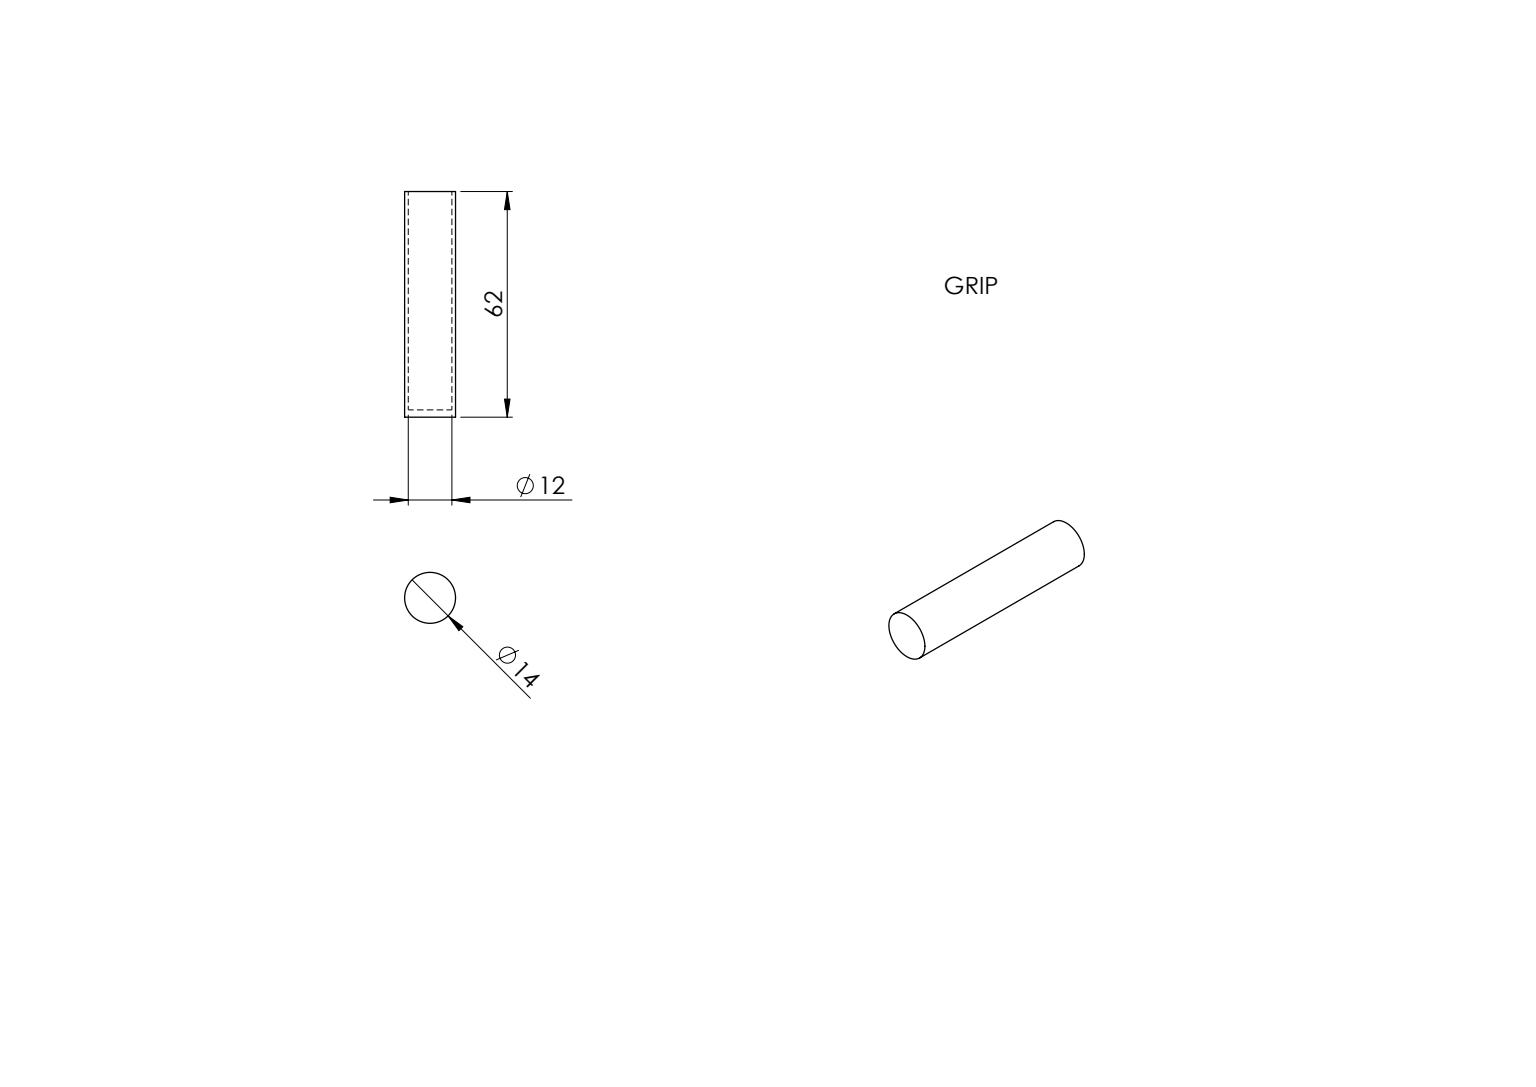
ISO-10303-21;
HEADER;
FILE_DESCRIPTION (('STEP AP214'),
    '1' );
FILE_NAME ('grip.step',
    '2026-10-25T17:17:34',
    ( '' ),
    ( '' ),
    'SwSTEP 2.0',
    'SolidWorks 2026',
    '' );
FILE_SCHEMA (( 'AUTOMOTIVE_DESIGN' ));
ENDSEC;

DATA;
#62=DIRECTION ( 'NONE',  ( -0.000000000000000000, -0.000000000000000000, -1.000000000000000000 ) ) ;
#172=ORIENTED_EDGE ( 'NONE', *, *, #15080, .F. ) ;
#270=PRODUCT_DEFINITION_CONTEXT ( 'detailed design', #8572, 'design' ) ;
#298=ORIENTED_EDGE ( 'NONE', *, *, #2474, .F. ) ;
#373=CARTESIAN_POINT ( 'NONE',  ( 118.5000000000000284, 12.69999999999998508, 50.00000000000001421 ) ) ;
#451=FACE_OUTER_BOUND ( 'NONE', #8763, .T. ) ;
#615=UNCERTAINTY_MEASURE_WITH_UNIT (LENGTH_MEASURE( 1.000000000000000082E-05 ), #15735, 'distance_accuracy_value', 'NONE');
#1092=MANIFOLD_SOLID_BREP ( 'Boss-Extrude1', #16920 ) ;
#1158=AXIS2_PLACEMENT_3D ( 'NONE', #12215, #18183, #17530 ) ;
#1175=( NAMED_UNIT ( * ) PLANE_ANGLE_UNIT ( ) SI_UNIT ( $, .RADIAN. ) );
#1608=EDGE_CURVE ( 'NONE', #14362, #14185, #5674, .T. ) ;
#1737=CIRCLE ( 'NONE', #11087, 7.000000000000006217 ) ;
#2052=SURFACE_STYLE_FILL_AREA ( #12504 ) ;
#2304=EDGE_CURVE ( 'NONE', #4985, #13752, #9705, .T. ) ;
#2362=CYLINDRICAL_SURFACE ( 'NONE', #4018, 6.000000000000005329 ) ;
#2377=AXIS2_PLACEMENT_3D ( 'NONE', #15410, #11206, #17171 ) ;
#2378=CARTESIAN_POINT ( 'NONE',  ( 111.5000000000000142, 12.69999999999998508, 50.00000000000001421 ) ) ;
#2402=VECTOR ( 'NONE', #3776, 1000.000000000000000 ) ;
#2444=FILL_AREA_STYLE_COLOUR ( '', #12359 ) ;
#2474=EDGE_CURVE ( 'NONE', #17401, #13752, #15823, .T. ) ;
#2675=ORIENTED_EDGE ( 'NONE', *, *, #1608, .F. ) ;
#2677=DIRECTION ( 'NONE',  ( 0.000000000000000000, 0.000000000000000000, 1.000000000000000000 ) ) ;
#2799=DIRECTION ( 'NONE',  ( 0.000000000000000000, 0.000000000000000000, 1.000000000000000000 ) ) ;
#2897=ORIENTED_EDGE ( 'NONE', *, *, #14345, .T. ) ;
#2959=PLANE ( 'NONE',  #16788 ) ;
#3036=CARTESIAN_POINT ( 'NONE',  ( 104.5000000000000142, 12.69999999999998508, 112.0000000000000142 ) ) ;
#3146=DIRECTION ( 'NONE',  ( 1.000000000000000000, 0.000000000000000000, -0.000000000000000000 ) ) ;
#3182=MECHANICAL_DESIGN_GEOMETRIC_PRESENTATION_REPRESENTATION('',(#3490),#12228);
#3285=CARTESIAN_POINT ( 'NONE',  ( 111.5000000000000142, 12.69999999999998508, 110.0000000000000142 ) ) ;
#3390=EDGE_CURVE ( 'NONE', #14362, #14762, #19288, .T. ) ;
#3398=CARTESIAN_POINT ( 'NONE',  ( 105.5000000000000142, 12.69999999999998508, 30.20101012677667285 ) ) ;
#3478=FACE_OUTER_BOUND ( 'NONE', #6668, .T. ) ;
#3490=STYLED_ITEM('',(#19371),#1092);
#3713=PRESENTATION_STYLE_ASSIGNMENT (( #17102 ) ) ;
#3732=DIRECTION ( 'NONE',  ( 0.000000000000000000, 0.000000000000000000, 1.000000000000000000 ) ) ;
#3776=DIRECTION ( 'NONE',  ( 0.000000000000000000, 0.000000000000000000, 1.000000000000000000 ) ) ;
#3898=PRODUCT_DEFINITION_SHAPE ( 'NONE', 'NONE',  #6427 ) ;
#3957=CARTESIAN_POINT ( 'NONE',  ( 111.5000000000000142, 12.69999999999998508, 112.0000000000000142 ) ) ;
#3973=AXIS2_PLACEMENT_3D ( 'NONE', #4322, #10283, #4415 ) ;
#4018=AXIS2_PLACEMENT_3D ( 'NONE', #9893, #3732, #9697 ) ;
#4056=EDGE_LOOP ( 'NONE', ( #9724, #11835, #9144, #298 ) ) ;
#4071=DIRECTION ( 'NONE',  ( -0.000000000000000000, -0.000000000000000000, -1.000000000000000000 ) ) ;
#4322=CARTESIAN_POINT ( 'NONE',  ( 111.5000000000000142, 12.69999999999998508, 50.00000000000001421 ) ) ;
#4415=DIRECTION ( 'NONE',  ( 1.000000000000000000, 0.000000000000000000, 0.000000000000000000 ) ) ;
#4603=DIRECTION ( 'NONE',  ( 0.000000000000000000, 0.000000000000000000, 1.000000000000000000 ) ) ;
#4840=ORIENTED_EDGE ( 'NONE', *, *, #7687, .T. ) ;
#4985=VERTEX_POINT ( 'NONE', #373 ) ;
#5072=SHAPE_DEFINITION_REPRESENTATION ( #3898, #7631 ) ;
#5095=SURFACE_SIDE_STYLE ('',( #2052 ) ) ;
#5102=UNCERTAINTY_MEASURE_WITH_UNIT (LENGTH_MEASURE( 1.000000000000000082E-05 ), #14163, 'distance_accuracy_value', 'NONE');
#5310=UNCERTAINTY_MEASURE_WITH_UNIT (LENGTH_MEASURE( 1.000000000000000082E-05 ), #9085, 'distance_accuracy_value', 'NONE');
#5540=VECTOR ( 'NONE', #11167, 1000.000000000000000 ) ;
#5545=ADVANCED_FACE ( 'NONE', ( #5770 ), #11721, .T. ) ;
#5674=LINE ( 'NONE', #17681, #6647 ) ;
#5770=FACE_OUTER_BOUND ( 'NONE', #4056, .T. ) ;
#5975=( NAMED_UNIT ( * ) PLANE_ANGLE_UNIT ( ) SI_UNIT ( $, .RADIAN. ) );
#6024=FACE_BOUND ( 'NONE', #16353, .T. ) ;
#6133=STYLED_ITEM ( 'NONE', ( #3713 ), #16944 ) ;
#6187=ORIENTED_EDGE ( 'NONE', *, *, #6983, .T. ) ;
#6284=ORIENTED_EDGE ( 'NONE', *, *, #12745, .T. ) ;
#6321=CIRCLE ( 'NONE', #17239, 6.000000000000005329 ) ;
#6397=ORIENTED_EDGE ( 'NONE', *, *, #3390, .F. ) ;
#6399=DIRECTION ( 'NONE',  ( 0.000000000000000000, 0.000000000000000000, 1.000000000000000000 ) ) ;
#6400=CARTESIAN_POINT ( 'NONE',  ( 111.5000000000000142, 12.69999999999998508, 50.00000000000001421 ) ) ;
#6427=PRODUCT_DEFINITION ( 'UNKNOWN', '', #7075, #270 ) ;
#6446=CIRCLE ( 'NONE', #13917, 6.000000000000005329 ) ;
#6495=ORIENTED_EDGE ( 'NONE', *, *, #14345, .F. ) ;
#6645=CIRCLE ( 'NONE', #17560, 7.000000000000006217 ) ;
#6647=VECTOR ( 'NONE', #8585, 1000.000000000000000 ) ;
#6668=EDGE_LOOP ( 'NONE', ( #8943, #6495 ) ) ;
#6782=ADVANCED_FACE ( 'NONE', ( #451 ), #11073, .T. ) ;
#6884=CARTESIAN_POINT ( 'NONE',  ( 111.5000000000000142, 12.69999999999998508, 30.20101012677667285 ) ) ;
#6983=EDGE_CURVE ( 'NONE', #4985, #14591, #6645, .T. ) ;
#7075=PRODUCT_DEFINITION_FORMATION_WITH_SPECIFIED_SOURCE ( 'ANY', '', #19045, .NOT_KNOWN. ) ;
#7341=CARTESIAN_POINT ( 'NONE',  ( 0.000000000000000000, 0.000000000000000000, 0.000000000000000000 ) ) ;
#7434=DIRECTION ( 'NONE',  ( 1.000000000000000000, 0.000000000000000000, 0.000000000000000000 ) ) ;
#7631=SHAPE_REPRESENTATION ( 'grip', ( #10540 ), #12052 ) ;
#7687=EDGE_CURVE ( 'NONE', #14185, #15086, #6321, .T. ) ;
#7713=AXIS2_PLACEMENT_3D ( 'NONE', #15862, #16627, #16433 ) ;
#7752=ORIENTED_EDGE ( 'NONE', *, *, #10666, .F. ) ;
#7817=CARTESIAN_POINT ( 'NONE',  ( 117.5000000000000142, 12.69999999999998508, 50.00000000000001421 ) ) ;
#7843=ORIENTED_EDGE ( 'NONE', *, *, #2474, .T. ) ;
#7983=VECTOR ( 'NONE', #18061, 1000.000000000000000 ) ;
#8018=ORIENTED_EDGE ( 'NONE', *, *, #11887, .T. ) ;
#8148=CARTESIAN_POINT ( 'NONE',  ( 111.5000000000000142, 12.69999999999998508, 30.20101012677667285 ) ) ;
#8361=CIRCLE ( 'NONE', #19292, 7.000000000000006217 ) ;
#8572=APPLICATION_CONTEXT ( 'automotive_design' ) ;
#8585=DIRECTION ( 'NONE',  ( 0.000000000000000000, 0.000000000000000000, 1.000000000000000000 ) ) ;
#8586=( NAMED_UNIT ( * ) SI_UNIT ( $, .STERADIAN. ) SOLID_ANGLE_UNIT ( ) );
#8688=EDGE_LOOP ( 'NONE', ( #172, #8018, #16737, #4840 ) ) ;
#8763=EDGE_LOOP ( 'NONE', ( #7752, #6284, #14948, #9162 ) ) ;
#8772=CARTESIAN_POINT ( 'NONE',  ( 104.5000000000000142, 12.69999999999998508, 30.20101012677667285 ) ) ;
#8862=LINE ( 'NONE', #8772, #7983 ) ;
#8943=ORIENTED_EDGE ( 'NONE', *, *, #7687, .F. ) ;
#8979=ORIENTED_EDGE ( 'NONE', *, *, #16774, .T. ) ;
#9017=CARTESIAN_POINT ( 'NONE',  ( 111.5000000000000142, 12.69999999999998508, 112.0000000000000142 ) ) ;
#9085=( LENGTH_UNIT ( ) NAMED_UNIT ( * ) SI_UNIT ( .MILLI., .METRE. ) );
#9144=ORIENTED_EDGE ( 'NONE', *, *, #2304, .T. ) ;
#9162=ORIENTED_EDGE ( 'NONE', *, *, #2304, .F. ) ;
#9345=CARTESIAN_POINT ( 'NONE',  ( 118.5000000000000284, 12.69999999999998508, 112.0000000000000142 ) ) ;
#9505=CARTESIAN_POINT ( 'NONE',  ( 118.5000000000000284, 12.69999999999998508, 30.20101012677667285 ) ) ;
#9617=DIRECTION ( 'NONE',  ( 1.000000000000000000, 0.000000000000000000, 0.000000000000000000 ) ) ;
#9697=DIRECTION ( 'NONE',  ( 1.000000000000000000, 0.000000000000000000, 0.000000000000000000 ) ) ;
#9705=LINE ( 'NONE', #9505, #5540 ) ;
#9724=ORIENTED_EDGE ( 'NONE', *, *, #12745, .F. ) ;
#9774=( NAMED_UNIT ( * ) SI_UNIT ( $, .STERADIAN. ) SOLID_ANGLE_UNIT ( ) );
#9893=CARTESIAN_POINT ( 'NONE',  ( 111.5000000000000142, 12.69999999999998508, 30.20101012677667285 ) ) ;
#10031=DIRECTION ( 'NONE',  ( 1.000000000000000000, 0.000000000000000000, 0.000000000000000000 ) ) ;
#10263=ORIENTED_EDGE ( 'NONE', *, *, #15080, .T. ) ;
#10283=DIRECTION ( 'NONE',  ( -0.000000000000000000, -0.000000000000000000, -1.000000000000000000 ) ) ;
#10460=( NAMED_UNIT ( * ) SI_UNIT ( $, .STERADIAN. ) SOLID_ANGLE_UNIT ( ) );
#10540=AXIS2_PLACEMENT_3D ( 'NONE', #7341, #19270, #11738 ) ;
#10666=EDGE_CURVE ( 'NONE', #14591, #4985, #1737, .T. ) ;
#10765=FACE_OUTER_BOUND ( 'NONE', #14570, .T. ) ;
#10770=ADVANCED_FACE ( 'NONE', ( #3478 ), #14031, .F. ) ;
#10999=DIRECTION ( 'NONE',  ( 1.000000000000000000, 0.000000000000000000, -0.000000000000000000 ) ) ;
#11073=CYLINDRICAL_SURFACE ( 'NONE', #18177, 7.000000000000006217 ) ;
#11087=AXIS2_PLACEMENT_3D ( 'NONE', #6400, #62, #15282 ) ;
#11167=DIRECTION ( 'NONE',  ( 0.000000000000000000, 0.000000000000000000, 1.000000000000000000 ) ) ;
#11206=DIRECTION ( 'NONE',  ( 0.000000000000000000, 0.000000000000000000, 1.000000000000000000 ) ) ;
#11289=ORIENTED_EDGE ( 'NONE', *, *, #10666, .T. ) ;
#11366=DIRECTION ( 'NONE',  ( 1.000000000000000000, 0.000000000000000000, 0.000000000000000000 ) ) ;
#11524=CARTESIAN_POINT ( 'NONE',  ( 105.5000000000000142, 12.69999999999998508, 50.00000000000001421 ) ) ;
#11704=ADVANCED_FACE ( 'NONE', ( #15508 ), #13937, .F. ) ;
#11721=CYLINDRICAL_SURFACE ( 'NONE', #12227, 7.000000000000006217 ) ;
#11732=( GEOMETRIC_REPRESENTATION_CONTEXT ( 3 ) GLOBAL_UNCERTAINTY_ASSIGNED_CONTEXT ( ( #5102 ) ) GLOBAL_UNIT_ASSIGNED_CONTEXT ( ( #14163, #1175, #8586 ) ) REPRESENTATION_CONTEXT ( 'NONE', 'WORKASPACE' ) );
#11738=DIRECTION ( 'NONE',  ( 1.000000000000000000, 0.000000000000000000, 0.000000000000000000 ) ) ;
#11835=ORIENTED_EDGE ( 'NONE', *, *, #6983, .F. ) ;
#11887=EDGE_CURVE ( 'NONE', #14762, #14362, #6446, .T. ) ;
#12019=CARTESIAN_POINT ( 'NONE',  ( 111.5000000000000142, 12.69999999999998508, 110.0000000000000142 ) ) ;
#12052=( GEOMETRIC_REPRESENTATION_CONTEXT ( 3 ) GLOBAL_UNCERTAINTY_ASSIGNED_CONTEXT ( ( #615 ) ) GLOBAL_UNIT_ASSIGNED_CONTEXT ( ( #15735, #17004, #9774 ) ) REPRESENTATION_CONTEXT ( 'NONE', 'WORKASPACE' ) );
#12215=CARTESIAN_POINT ( 'NONE',  ( 111.5000000000000142, 12.69999999999998508, 110.0000000000000142 ) ) ;
#12227=AXIS2_PLACEMENT_3D ( 'NONE', #6884, #17329, #9617 ) ;
#12228=( GEOMETRIC_REPRESENTATION_CONTEXT ( 3 ) GLOBAL_UNCERTAINTY_ASSIGNED_CONTEXT ( ( #5310 ) ) GLOBAL_UNIT_ASSIGNED_CONTEXT ( ( #9085, #5975, #10460 ) ) REPRESENTATION_CONTEXT ( 'NONE', 'WORKASPACE' ) );
#12359=COLOUR_RGB ( '',0.8941176470588234615, 0.8941176470588234615, 0.8941176470588234615 ) ;
#12500=CARTESIAN_POINT ( 'NONE',  ( 104.5000000000000142, 12.69999999999998508, 50.00000000000001421 ) ) ;
#12504=FILL_AREA_STYLE ('',( #2444 ) ) ;
#12666=CARTESIAN_POINT ( 'NONE',  ( 105.5000000000000142, 12.69999999999998508, 110.0000000000000142 ) ) ;
#12745=EDGE_CURVE ( 'NONE', #14591, #17401, #8862, .T. ) ;
#13307=ADVANCED_FACE ( 'NONE', ( #10765 ), #2959, .T. ) ;
#13413=DIRECTION ( 'NONE',  ( 0.000000000000000000, 0.000000000000000000, 1.000000000000000000 ) ) ;
#13435=CARTESIAN_POINT ( 'NONE',  ( 117.5000000000000142, 12.69999999999998508, 110.0000000000000142 ) ) ;
#13620=CIRCLE ( 'NONE', #1158, 6.000000000000005329 ) ;
#13752=VERTEX_POINT ( 'NONE', #9345 ) ;
#13917=AXIS2_PLACEMENT_3D ( 'NONE', #17553, #4071, #10031 ) ;
#13930=DIRECTION ( 'NONE',  ( 0.000000000000000000, 0.000000000000000000, 1.000000000000000000 ) ) ;
#13937=CYLINDRICAL_SURFACE ( 'NONE', #2377, 6.000000000000005329 ) ;
#13945=PRODUCT_CONTEXT ( 'NONE', #18425, 'mechanical' ) ;
#14031=PLANE ( 'NONE',  #14512 ) ;
#14099=DIRECTION ( 'NONE',  ( 1.000000000000000000, 0.000000000000000000, 0.000000000000000000 ) ) ;
#14163=( LENGTH_UNIT ( ) NAMED_UNIT ( * ) SI_UNIT ( .MILLI., .METRE. ) );
#14185=VERTEX_POINT ( 'NONE', #13435 ) ;
#14279=FACE_OUTER_BOUND ( 'NONE', #8688, .T. ) ;
#14345=EDGE_CURVE ( 'NONE', #15086, #14185, #13620, .T. ) ;
#14362=VERTEX_POINT ( 'NONE', #7817 ) ;
#14512=AXIS2_PLACEMENT_3D ( 'NONE', #3285, #13930, #10999 ) ;
#14570=EDGE_LOOP ( 'NONE', ( #8979, #7843 ) ) ;
#14572=DIRECTION ( 'NONE',  ( -0.000000000000000000, -0.000000000000000000, -1.000000000000000000 ) ) ;
#14591=VERTEX_POINT ( 'NONE', #12500 ) ;
#14762=VERTEX_POINT ( 'NONE', #11524 ) ;
#14905=DIRECTION ( 'NONE',  ( 1.000000000000000000, 0.000000000000000000, -0.000000000000000000 ) ) ;
#14948=ORIENTED_EDGE ( 'NONE', *, *, #16774, .F. ) ;
#15036=ORIENTED_EDGE ( 'NONE', *, *, #3390, .T. ) ;
#15080=EDGE_CURVE ( 'NONE', #14762, #15086, #15218, .T. ) ;
#15086=VERTEX_POINT ( 'NONE', #12666 ) ;
#15098=PLANE ( 'NONE',  #16149 ) ;
#15218=LINE ( 'NONE', #3398, #2402 ) ;
#15282=DIRECTION ( 'NONE',  ( 1.000000000000000000, 0.000000000000000000, 0.000000000000000000 ) ) ;
#15410=CARTESIAN_POINT ( 'NONE',  ( 111.5000000000000142, 12.69999999999998508, 30.20101012677667285 ) ) ;
#15508=FACE_OUTER_BOUND ( 'NONE', #18968, .T. ) ;
#15576=ADVANCED_FACE ( 'NONE', ( #16191, #6024 ), #15098, .F. ) ;
#15735=( LENGTH_UNIT ( ) NAMED_UNIT ( * ) SI_UNIT ( .MILLI., .METRE. ) );
#15823=CIRCLE ( 'NONE', #7713, 7.000000000000006217 ) ;
#15862=CARTESIAN_POINT ( 'NONE',  ( 111.5000000000000142, 12.69999999999998508, 112.0000000000000142 ) ) ;
#15884=DIRECTION ( 'NONE',  ( 1.000000000000000000, 0.000000000000000000, 0.000000000000000000 ) ) ;
#16027=EDGE_LOOP ( 'NONE', ( #6187, #11289 ) ) ;
#16149=AXIS2_PLACEMENT_3D ( 'NONE', #16375, #2799, #14905 ) ;
#16191=FACE_OUTER_BOUND ( 'NONE', #16027, .T. ) ;
#16222=SHAPE_REPRESENTATION_RELATIONSHIP ( 'NONE' , 'NONE' ,  #7631, #16944 ) ;
#16353=EDGE_LOOP ( 'NONE', ( #6397, #18776 ) ) ;
#16375=CARTESIAN_POINT ( 'NONE',  ( 111.5000000000000142, 12.69999999999998508, 50.00000000000001421 ) ) ;
#16433=DIRECTION ( 'NONE',  ( 1.000000000000000000, 0.000000000000000000, 0.000000000000000000 ) ) ;
#16627=DIRECTION ( 'NONE',  ( 0.000000000000000000, 0.000000000000000000, 1.000000000000000000 ) ) ;
#16737=ORIENTED_EDGE ( 'NONE', *, *, #1608, .T. ) ;
#16774=EDGE_CURVE ( 'NONE', #13752, #17401, #8361, .T. ) ;
#16788=AXIS2_PLACEMENT_3D ( 'NONE', #9017, #13413, #3146 ) ;
#16920=CLOSED_SHELL ( 'NONE', ( #11704, #6782, #5545, #18323, #15576, #10770, #13307 ) ) ;
#16944=ADVANCED_BREP_SHAPE_REPRESENTATION ( '', ( #1092, #10540 ), #12052 ) ;
#17004=( NAMED_UNIT ( * ) PLANE_ANGLE_UNIT ( ) SI_UNIT ( $, .RADIAN. ) );
#17102=SURFACE_STYLE_USAGE ( .BOTH. , #5095 ) ;
#17171=DIRECTION ( 'NONE',  ( 1.000000000000000000, 0.000000000000000000, 0.000000000000000000 ) ) ;
#17239=AXIS2_PLACEMENT_3D ( 'NONE', #12019, #4603, #7434 ) ;
#17329=DIRECTION ( 'NONE',  ( 0.000000000000000000, 0.000000000000000000, 1.000000000000000000 ) ) ;
#17401=VERTEX_POINT ( 'NONE', #3036 ) ;
#17530=DIRECTION ( 'NONE',  ( 1.000000000000000000, 0.000000000000000000, 0.000000000000000000 ) ) ;
#17553=CARTESIAN_POINT ( 'NONE',  ( 111.5000000000000142, 12.69999999999998508, 50.00000000000001421 ) ) ;
#17560=AXIS2_PLACEMENT_3D ( 'NONE', #2378, #14572, #11366 ) ;
#17681=CARTESIAN_POINT ( 'NONE',  ( 117.5000000000000142, 12.69999999999998508, 30.20101012677667285 ) ) ;
#18061=DIRECTION ( 'NONE',  ( 0.000000000000000000, 0.000000000000000000, 1.000000000000000000 ) ) ;
#18177=AXIS2_PLACEMENT_3D ( 'NONE', #8148, #6399, #14099 ) ;
#18183=DIRECTION ( 'NONE',  ( 0.000000000000000000, 0.000000000000000000, 1.000000000000000000 ) ) ;
#18297=MECHANICAL_DESIGN_GEOMETRIC_PRESENTATION_REPRESENTATION('',(#6133),#11732);
#18323=ADVANCED_FACE ( 'NONE', ( #14279 ), #2362, .F. ) ;
#18425=APPLICATION_CONTEXT ( 'automotive_design' ) ;
#18776=ORIENTED_EDGE ( 'NONE', *, *, #11887, .F. ) ;
#18968=EDGE_LOOP ( 'NONE', ( #15036, #10263, #2897, #2675 ) ) ;
#19045=PRODUCT ( 'grip', 'grip', '', ( #13945 ) ) ;
#19270=DIRECTION ( 'NONE',  ( 0.000000000000000000, 0.000000000000000000, 1.000000000000000000 ) ) ;
#19288=CIRCLE ( 'NONE', #3973, 6.000000000000005329 ) ;
#19292=AXIS2_PLACEMENT_3D ( 'NONE', #3957, #2677, #15884 ) ;
#19365=COLOUR_RGB('Black',0.12,0.14,0.17);
#19366=FILL_AREA_STYLE_COLOUR('',#19365);
#19367=FILL_AREA_STYLE('',(#19366));
#19368=SURFACE_STYLE_FILL_AREA(#19367);
#19369=SURFACE_SIDE_STYLE('',(#19368));
#19370=SURFACE_STYLE_USAGE(.BOTH.,#19369);
#19371=PRESENTATION_STYLE_ASSIGNMENT((#19370));
ENDSEC;
END-ISO-10303-21;
